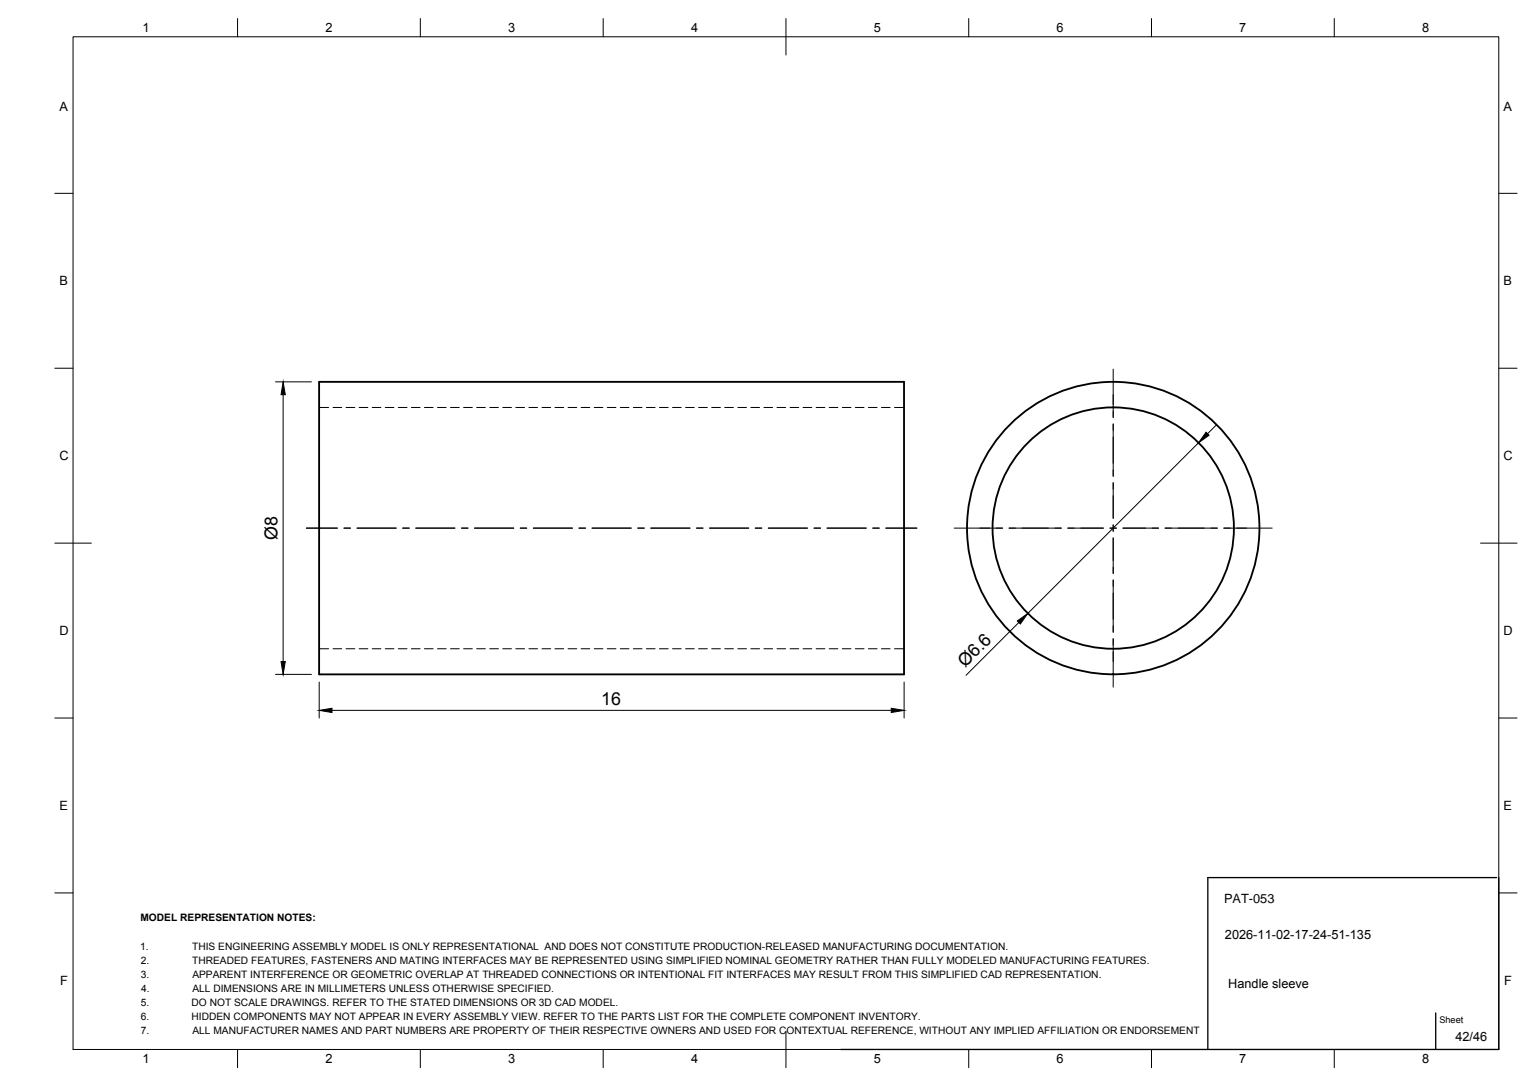
ISO-10303-21;
HEADER;
/* Generated by software containing ST-Developer
 * from STEP Tools, Inc. (www.steptools.com) 
 */

FILE_DESCRIPTION(
/* description */ ('Hand-operated arbor press'),
/* implementation_level */ '2;1');

FILE_NAME(
/* name */ 'Handle sleeve.step',
/* time_stamp */ '2026-10-28T03:25:25-07:00',
/* author */ (''),
/* organization */ (''),
/* preprocessor_version */ 'ST-DEVELOPER v20.2',
/* originating_system */ 'Autodesk Translation Framework v15.17.0.0',
/* authorisation */ '');

FILE_SCHEMA (('AUTOMOTIVE_DESIGN { 1 0 10303 214 3 1 1 }'));
ENDSEC;

DATA;
#10=MECHANICAL_DESIGN_GEOMETRIC_PRESENTATION_REPRESENTATION('',(#627),#32751);
#536=SHAPE_REPRESENTATION_RELATIONSHIP('SRR','None',#32968,#578);
#578=ADVANCED_BREP_SHAPE_REPRESENTATION('',(#674),#32742);
#627=STYLED_ITEM('',(#33256),#674);
#674=MANIFOLD_SOLID_BREP('Body1',#12526);
#834=FACE_BOUND('',#2670,.T.);
#835=FACE_BOUND('',#2672,.T.);
#1235=PLANE('',#13903);
#1236=PLANE('',#13904);
#1832=FACE_OUTER_BOUND('',#2667,.T.);
#1833=FACE_OUTER_BOUND('',#2668,.T.);
#1834=FACE_OUTER_BOUND('',#2669,.T.);
#1835=FACE_OUTER_BOUND('',#2671,.T.);
#2667=EDGE_LOOP('',(#10944,#10945,#10946,#10947));
#2668=EDGE_LOOP('',(#10948,#10949,#10950,#10951));
#2669=EDGE_LOOP('',(#10952));
#2670=EDGE_LOOP('',(#10953));
#2671=EDGE_LOOP('',(#10954));
#2672=EDGE_LOOP('',(#10955));
#3806=LINE('',#20781,#4977);
#3807=LINE('',#20787,#4978);
#4977=VECTOR('',#16937,0.33);
#4978=VECTOR('',#16944,0.4);
#5476=CIRCLE('',#13898,0.33);
#5477=CIRCLE('',#13899,0.33);
#5478=CIRCLE('',#13901,0.4);
#5479=CIRCLE('',#13902,0.4);
#6435=VERTEX_POINT('',#20778);
#6436=VERTEX_POINT('',#20780);
#6437=VERTEX_POINT('',#20784);
#6438=VERTEX_POINT('',#20786);
#7975=EDGE_CURVE('',#6435,#6435,#5476,.T.);
#7976=EDGE_CURVE('',#6435,#6436,#3806,.T.);
#7977=EDGE_CURVE('',#6436,#6436,#5477,.T.);
#7978=EDGE_CURVE('',#6437,#6437,#5478,.T.);
#7979=EDGE_CURVE('',#6437,#6438,#3807,.T.);
#7980=EDGE_CURVE('',#6438,#6438,#5479,.T.);
#10944=ORIENTED_EDGE('',*,*,#7975,.F.);
#10945=ORIENTED_EDGE('',*,*,#7976,.T.);
#10946=ORIENTED_EDGE('',*,*,#7977,.T.);
#10947=ORIENTED_EDGE('',*,*,#7976,.F.);
#10948=ORIENTED_EDGE('',*,*,#7978,.F.);
#10949=ORIENTED_EDGE('',*,*,#7979,.T.);
#10950=ORIENTED_EDGE('',*,*,#7980,.T.);
#10951=ORIENTED_EDGE('',*,*,#7979,.F.);
#10952=ORIENTED_EDGE('',*,*,#7978,.T.);
#10953=ORIENTED_EDGE('',*,*,#7975,.T.);
#10954=ORIENTED_EDGE('',*,*,#7980,.F.);
#10955=ORIENTED_EDGE('',*,*,#7977,.F.);
#11766=CYLINDRICAL_SURFACE('',#13897,0.33);
#11767=CYLINDRICAL_SURFACE('',#13900,0.4);
#12341=ADVANCED_FACE('',(#1832),#11766,.F.);
#12342=ADVANCED_FACE('',(#1833),#11767,.T.);
#12343=ADVANCED_FACE('',(#1834,#834),#1235,.T.);
#12344=ADVANCED_FACE('',(#1835,#835),#1236,.F.);
#12526=CLOSED_SHELL('',(#12341,#12342,#12343,#12344));
#13896=AXIS2_PLACEMENT_3D('',#20776,#16931,#16932);
#13897=AXIS2_PLACEMENT_3D('',#20777,#16933,#16934);
#13898=AXIS2_PLACEMENT_3D('',#20779,#16935,#16936);
#13899=AXIS2_PLACEMENT_3D('',#20782,#16938,#16939);
#13900=AXIS2_PLACEMENT_3D('',#20783,#16940,#16941);
#13901=AXIS2_PLACEMENT_3D('',#20785,#16942,#16943);
#13902=AXIS2_PLACEMENT_3D('',#20788,#16945,#16946);
#13903=AXIS2_PLACEMENT_3D('',#20789,#16947,#16948);
#13904=AXIS2_PLACEMENT_3D('',#20790,#16949,#16950);
#16931=DIRECTION('axis',(0.,0.,1.));
#16932=DIRECTION('refdir',(1.,0.,0.));
#16933=DIRECTION('center_axis',(0.,1.,0.));
#16934=DIRECTION('ref_axis',(1.,0.,0.));
#16935=DIRECTION('center_axis',(0.,-1.,0.));
#16936=DIRECTION('ref_axis',(1.,0.,0.));
#16937=DIRECTION('',(0.,-1.,0.));
#16938=DIRECTION('center_axis',(0.,-1.,0.));
#16939=DIRECTION('ref_axis',(1.,0.,0.));
#16940=DIRECTION('center_axis',(0.,1.,0.));
#16941=DIRECTION('ref_axis',(1.,0.,0.));
#16942=DIRECTION('center_axis',(0.,1.,0.));
#16943=DIRECTION('ref_axis',(1.,0.,0.));
#16944=DIRECTION('',(0.,-1.,0.));
#16945=DIRECTION('center_axis',(0.,1.,0.));
#16946=DIRECTION('ref_axis',(1.,0.,0.));
#16947=DIRECTION('center_axis',(0.,1.,0.));
#16948=DIRECTION('ref_axis',(1.,0.,0.));
#16949=DIRECTION('center_axis',(0.,1.,0.));
#16950=DIRECTION('ref_axis',(1.,0.,0.));
#20776=CARTESIAN_POINT('',(0.,0.,0.));
#20777=CARTESIAN_POINT('Origin',(-3.25,6.8,29.));
#20778=CARTESIAN_POINT('',(-3.58,8.4,29.));
#20779=CARTESIAN_POINT('Origin',(-3.25,8.4,29.));
#20780=CARTESIAN_POINT('',(-3.58,6.8,29.));
#20781=CARTESIAN_POINT('',(-3.58,6.8,29.));
#20782=CARTESIAN_POINT('Origin',(-3.25,6.8,29.));
#20783=CARTESIAN_POINT('Origin',(-3.25,6.8,29.));
#20784=CARTESIAN_POINT('',(-3.65,8.4,29.));
#20785=CARTESIAN_POINT('Origin',(-3.25,8.4,29.));
#20786=CARTESIAN_POINT('',(-3.65,6.8,29.));
#20787=CARTESIAN_POINT('',(-3.65,6.8,29.));
#20788=CARTESIAN_POINT('Origin',(-3.25,6.8,29.));
#20789=CARTESIAN_POINT('Origin',(-3.25,8.4,29.));
#20790=CARTESIAN_POINT('Origin',(-3.25,6.8,29.));
#32693=UNCERTAINTY_MEASURE_WITH_UNIT(LENGTH_MEASURE(0.001),#32752,
'DISTANCE_ACCURACY_VALUE',
'Maximum model space distance between geometric entities at asserted c
onnectivities');
#32702=UNCERTAINTY_MEASURE_WITH_UNIT(LENGTH_MEASURE(0.001),#32752,
'DISTANCE_ACCURACY_VALUE',
'Maximum model space distance between geometric entities at asserted c
onnectivities');
#32742=(
GEOMETRIC_REPRESENTATION_CONTEXT(3)
GLOBAL_UNCERTAINTY_ASSIGNED_CONTEXT((#32693))
GLOBAL_UNIT_ASSIGNED_CONTEXT((#32752,#32754,#32755))
REPRESENTATION_CONTEXT('','3D')
);
#32751=(
GEOMETRIC_REPRESENTATION_CONTEXT(3)
GLOBAL_UNCERTAINTY_ASSIGNED_CONTEXT((#32702))
GLOBAL_UNIT_ASSIGNED_CONTEXT((#32752,#32754,#32755))
REPRESENTATION_CONTEXT('','3D')
);
#32752=(
LENGTH_UNIT()
NAMED_UNIT(*)
SI_UNIT(.CENTI.,.METRE.)
);
#32754=(
NAMED_UNIT(*)
PLANE_ANGLE_UNIT()
SI_UNIT($,.RADIAN.)
);
#32755=(
NAMED_UNIT(*)
SI_UNIT($,.STERADIAN.)
SOLID_ANGLE_UNIT()
);
#32795=SHAPE_DEFINITION_REPRESENTATION(#32852,#32968);
#32852=PRODUCT_DEFINITION_SHAPE('',$,#33017);
#32968=SHAPE_REPRESENTATION('',(#13896),#32742);
#32977=PRODUCT_DEFINITION_CONTEXT('part definition',#33123,'design');
#33017=PRODUCT_DEFINITION('Handle sleeve','Handle sleeve',#33065,#32977);
#33065=PRODUCT_DEFINITION_FORMATION('',$,#33164);
#33123=APPLICATION_CONTEXT(
'Core Data for Automotive Mechanical Design Process');
#33124=PRODUCT_CONTEXT('part definition',#33123,'mechanical');
#33164=PRODUCT('Handle sleeve','Handle sleeve','Handle sleeve',(#33124));
#33250=COLOUR_RGB('Off White',0.89,0.88,0.83);
#33251=FILL_AREA_STYLE_COLOUR('',#33250);
#33252=FILL_AREA_STYLE('',(#33251));
#33253=SURFACE_STYLE_FILL_AREA(#33252);
#33254=SURFACE_SIDE_STYLE('',(#33253));
#33255=SURFACE_STYLE_USAGE(.BOTH.,#33254);
#33256=PRESENTATION_STYLE_ASSIGNMENT((#33255));
ENDSEC;
END-ISO-10303-21;
